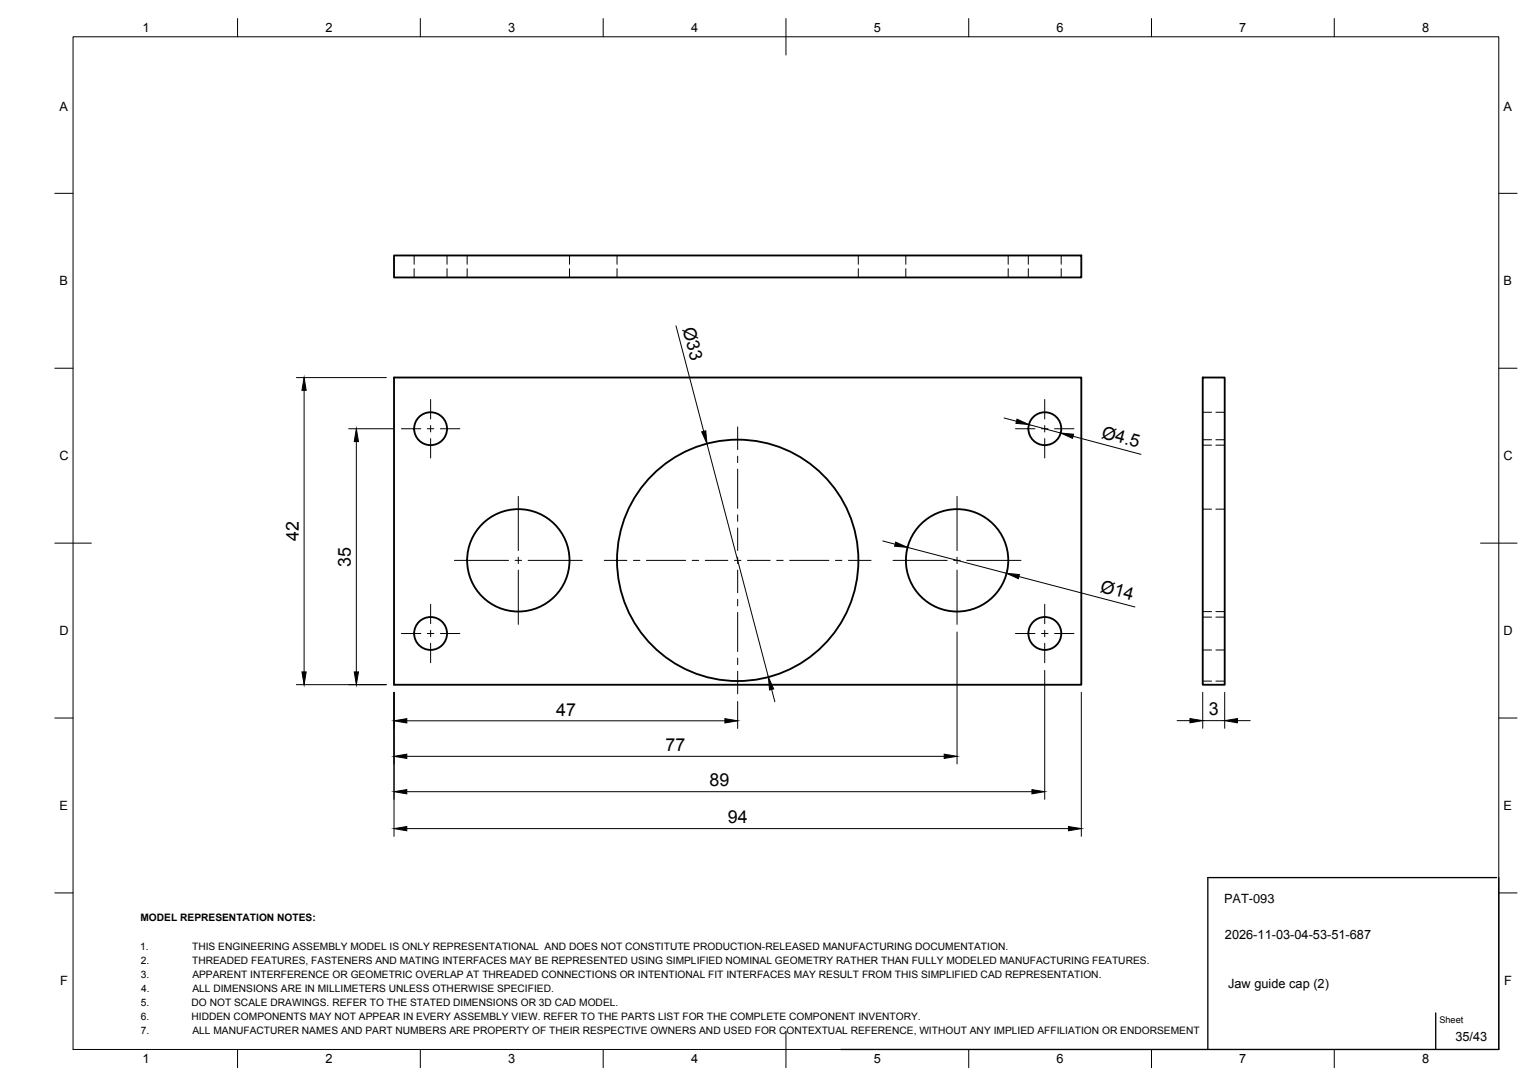
ISO-10303-21;
HEADER;
/* Generated by software containing ST-Developer
 * from STEP Tools, Inc. (www.steptools.com) 
 */

FILE_DESCRIPTION(
/* description */ ('Self-centering screw clamp'),
/* implementation_level */ '2;1');

FILE_NAME(
/* name */ 'Jaw guide cap (2).step',
/* time_stamp */ '2026-10-28T03:25:31-07:00',
/* author */ (''),
/* organization */ (''),
/* preprocessor_version */ 'ST-DEVELOPER v20.2',
/* originating_system */ 'Autodesk Translation Framework v15.17.0.0',
/* authorisation */ '');

FILE_SCHEMA (('AUTOMOTIVE_DESIGN { 1 0 10303 214 3 1 1 }'));
ENDSEC;

DATA;
#10=MECHANICAL_DESIGN_GEOMETRIC_PRESENTATION_REPRESENTATION('',(#656),#16799);
#567=SHAPE_REPRESENTATION_RELATIONSHIP('SRR','None',#17043,#608);
#608=ADVANCED_BREP_SHAPE_REPRESENTATION('',(#704),#16781);
#656=STYLED_ITEM('',(#17312),#704);
#704=MANIFOLD_SOLID_BREP('Body1',#9107);
#936=FACE_BOUND('',#2337,.T.);
#937=FACE_BOUND('',#2338,.T.);
#938=FACE_BOUND('',#2339,.T.);
#939=FACE_BOUND('',#2340,.T.);
#940=FACE_BOUND('',#2341,.T.);
#941=FACE_BOUND('',#2342,.T.);
#942=FACE_BOUND('',#2343,.T.);
#943=FACE_BOUND('',#2346,.T.);
#944=FACE_BOUND('',#2347,.T.);
#945=FACE_BOUND('',#2348,.T.);
#946=FACE_BOUND('',#2349,.T.);
#947=FACE_BOUND('',#2350,.T.);
#948=FACE_BOUND('',#2351,.T.);
#949=FACE_BOUND('',#2352,.T.);
#1173=PLANE('',#10330);
#1174=PLANE('',#10331);
#1175=PLANE('',#10332);
#1176=PLANE('',#10333);
#1177=PLANE('',#10334);
#1178=PLANE('',#10335);
#1606=FACE_OUTER_BOUND('',#2328,.T.);
#1607=FACE_OUTER_BOUND('',#2329,.T.);
#1608=FACE_OUTER_BOUND('',#2330,.T.);
#1609=FACE_OUTER_BOUND('',#2331,.T.);
#1610=FACE_OUTER_BOUND('',#2332,.T.);
#1611=FACE_OUTER_BOUND('',#2333,.T.);
#1612=FACE_OUTER_BOUND('',#2334,.T.);
#1613=FACE_OUTER_BOUND('',#2335,.T.);
#1614=FACE_OUTER_BOUND('',#2336,.T.);
#1615=FACE_OUTER_BOUND('',#2344,.T.);
#1616=FACE_OUTER_BOUND('',#2345,.T.);
#1617=FACE_OUTER_BOUND('',#2353,.T.);
#1618=FACE_OUTER_BOUND('',#2354,.T.);
#2328=EDGE_LOOP('',(#7653,#7654,#7655,#7656));
#2329=EDGE_LOOP('',(#7657,#7658,#7659,#7660));
#2330=EDGE_LOOP('',(#7661,#7662,#7663,#7664));
#2331=EDGE_LOOP('',(#7665,#7666,#7667,#7668));
#2332=EDGE_LOOP('',(#7669,#7670,#7671,#7672));
#2333=EDGE_LOOP('',(#7673,#7674,#7675,#7676));
#2334=EDGE_LOOP('',(#7677,#7678,#7679,#7680));
#2335=EDGE_LOOP('',(#7681,#7682,#7683,#7684));
#2336=EDGE_LOOP('',(#7685,#7686,#7687,#7688));
#2337=EDGE_LOOP('',(#7689));
#2338=EDGE_LOOP('',(#7690));
#2339=EDGE_LOOP('',(#7691));
#2340=EDGE_LOOP('',(#7692));
#2341=EDGE_LOOP('',(#7693));
#2342=EDGE_LOOP('',(#7694));
#2343=EDGE_LOOP('',(#7695));
#2344=EDGE_LOOP('',(#7696,#7697,#7698,#7699));
#2345=EDGE_LOOP('',(#7700,#7701,#7702,#7703));
#2346=EDGE_LOOP('',(#7704));
#2347=EDGE_LOOP('',(#7705));
#2348=EDGE_LOOP('',(#7706));
#2349=EDGE_LOOP('',(#7707));
#2350=EDGE_LOOP('',(#7708));
#2351=EDGE_LOOP('',(#7709));
#2352=EDGE_LOOP('',(#7710));
#2353=EDGE_LOOP('',(#7711,#7712,#7713,#7714));
#2354=EDGE_LOOP('',(#7715,#7716,#7717,#7718));
#2959=LINE('',#15709,#3532);
#2960=LINE('',#15715,#3533);
#2961=LINE('',#15721,#3534);
#2962=LINE('',#15727,#3535);
#2963=LINE('',#15733,#3536);
#2964=LINE('',#15739,#3537);
#2965=LINE('',#15745,#3538);
#2966=LINE('',#15750,#3539);
#2967=LINE('',#15752,#3540);
#2968=LINE('',#15754,#3541);
#2969=LINE('',#15755,#3542);
#2970=LINE('',#15758,#3543);
#2971=LINE('',#15760,#3544);
#2972=LINE('',#15761,#3545);
#2973=LINE('',#15764,#3546);
#2974=LINE('',#15766,#3547);
#2975=LINE('',#15767,#3548);
#2976=LINE('',#15769,#3549);
#2977=LINE('',#15770,#3550);
#3532=VECTOR('',#12602,0.225);
#3533=VECTOR('',#12609,0.225);
#3534=VECTOR('',#12616,0.225);
#3535=VECTOR('',#12623,0.225);
#3536=VECTOR('',#12630,1.65);
#3537=VECTOR('',#12637,0.7);
#3538=VECTOR('',#12644,0.7);
#3539=VECTOR('',#12649,1.);
#3540=VECTOR('',#12650,1.);
#3541=VECTOR('',#12651,1.);
#3542=VECTOR('',#12652,1.);
#3543=VECTOR('',#12655,1.);
#3544=VECTOR('',#12656,1.);
#3545=VECTOR('',#12657,1.);
#3546=VECTOR('',#12660,1.);
#3547=VECTOR('',#12661,1.);
#3548=VECTOR('',#12662,1.);
#3549=VECTOR('',#12665,1.);
#3550=VECTOR('',#12666,1.);
#4086=CIRCLE('',#10310,0.225);
#4087=CIRCLE('',#10311,0.225);
#4088=CIRCLE('',#10313,0.225);
#4089=CIRCLE('',#10314,0.225);
#4090=CIRCLE('',#10316,0.225);
#4091=CIRCLE('',#10317,0.225);
#4092=CIRCLE('',#10319,0.225);
#4093=CIRCLE('',#10320,0.225);
#4094=CIRCLE('',#10322,1.65);
#4095=CIRCLE('',#10323,1.65);
#4096=CIRCLE('',#10325,0.7);
#4097=CIRCLE('',#10326,0.7);
#4098=CIRCLE('',#10328,0.7);
#4099=CIRCLE('',#10329,0.7);
#4745=VERTEX_POINT('',#15706);
#4746=VERTEX_POINT('',#15708);
#4747=VERTEX_POINT('',#15712);
#4748=VERTEX_POINT('',#15714);
#4749=VERTEX_POINT('',#15718);
#4750=VERTEX_POINT('',#15720);
#4751=VERTEX_POINT('',#15724);
#4752=VERTEX_POINT('',#15726);
#4753=VERTEX_POINT('',#15730);
#4754=VERTEX_POINT('',#15732);
#4755=VERTEX_POINT('',#15736);
#4756=VERTEX_POINT('',#15738);
#4757=VERTEX_POINT('',#15742);
#4758=VERTEX_POINT('',#15744);
#4759=VERTEX_POINT('',#15748);
#4760=VERTEX_POINT('',#15749);
#4761=VERTEX_POINT('',#15751);
#4762=VERTEX_POINT('',#15753);
#4763=VERTEX_POINT('',#15757);
#4764=VERTEX_POINT('',#15759);
#4765=VERTEX_POINT('',#15763);
#4766=VERTEX_POINT('',#15765);
#5751=EDGE_CURVE('',#4745,#4745,#4086,.T.);
#5752=EDGE_CURVE('',#4745,#4746,#2959,.T.);
#5753=EDGE_CURVE('',#4746,#4746,#4087,.T.);
#5754=EDGE_CURVE('',#4747,#4747,#4088,.T.);
#5755=EDGE_CURVE('',#4747,#4748,#2960,.T.);
#5756=EDGE_CURVE('',#4748,#4748,#4089,.T.);
#5757=EDGE_CURVE('',#4749,#4749,#4090,.T.);
#5758=EDGE_CURVE('',#4749,#4750,#2961,.T.);
#5759=EDGE_CURVE('',#4750,#4750,#4091,.T.);
#5760=EDGE_CURVE('',#4751,#4751,#4092,.T.);
#5761=EDGE_CURVE('',#4751,#4752,#2962,.T.);
#5762=EDGE_CURVE('',#4752,#4752,#4093,.T.);
#5763=EDGE_CURVE('',#4753,#4753,#4094,.T.);
#5764=EDGE_CURVE('',#4753,#4754,#2963,.T.);
#5765=EDGE_CURVE('',#4754,#4754,#4095,.T.);
#5766=EDGE_CURVE('',#4755,#4755,#4096,.T.);
#5767=EDGE_CURVE('',#4755,#4756,#2964,.T.);
#5768=EDGE_CURVE('',#4756,#4756,#4097,.T.);
#5769=EDGE_CURVE('',#4757,#4757,#4098,.T.);
#5770=EDGE_CURVE('',#4757,#4758,#2965,.T.);
#5771=EDGE_CURVE('',#4758,#4758,#4099,.T.);
#5772=EDGE_CURVE('',#4759,#4760,#2966,.T.);
#5773=EDGE_CURVE('',#4760,#4761,#2967,.T.);
#5774=EDGE_CURVE('',#4762,#4761,#2968,.T.);
#5775=EDGE_CURVE('',#4759,#4762,#2969,.T.);
#5776=EDGE_CURVE('',#4763,#4759,#2970,.T.);
#5777=EDGE_CURVE('',#4764,#4762,#2971,.T.);
#5778=EDGE_CURVE('',#4763,#4764,#2972,.T.);
#5779=EDGE_CURVE('',#4765,#4763,#2973,.T.);
#5780=EDGE_CURVE('',#4766,#4764,#2974,.T.);
#5781=EDGE_CURVE('',#4765,#4766,#2975,.T.);
#5782=EDGE_CURVE('',#4760,#4765,#2976,.T.);
#5783=EDGE_CURVE('',#4761,#4766,#2977,.T.);
#7653=ORIENTED_EDGE('',*,*,#5751,.F.);
#7654=ORIENTED_EDGE('',*,*,#5752,.T.);
#7655=ORIENTED_EDGE('',*,*,#5753,.F.);
#7656=ORIENTED_EDGE('',*,*,#5752,.F.);
#7657=ORIENTED_EDGE('',*,*,#5754,.F.);
#7658=ORIENTED_EDGE('',*,*,#5755,.T.);
#7659=ORIENTED_EDGE('',*,*,#5756,.F.);
#7660=ORIENTED_EDGE('',*,*,#5755,.F.);
#7661=ORIENTED_EDGE('',*,*,#5757,.F.);
#7662=ORIENTED_EDGE('',*,*,#5758,.T.);
#7663=ORIENTED_EDGE('',*,*,#5759,.F.);
#7664=ORIENTED_EDGE('',*,*,#5758,.F.);
#7665=ORIENTED_EDGE('',*,*,#5760,.F.);
#7666=ORIENTED_EDGE('',*,*,#5761,.T.);
#7667=ORIENTED_EDGE('',*,*,#5762,.F.);
#7668=ORIENTED_EDGE('',*,*,#5761,.F.);
#7669=ORIENTED_EDGE('',*,*,#5763,.F.);
#7670=ORIENTED_EDGE('',*,*,#5764,.T.);
#7671=ORIENTED_EDGE('',*,*,#5765,.F.);
#7672=ORIENTED_EDGE('',*,*,#5764,.F.);
#7673=ORIENTED_EDGE('',*,*,#5766,.F.);
#7674=ORIENTED_EDGE('',*,*,#5767,.T.);
#7675=ORIENTED_EDGE('',*,*,#5768,.F.);
#7676=ORIENTED_EDGE('',*,*,#5767,.F.);
#7677=ORIENTED_EDGE('',*,*,#5769,.F.);
#7678=ORIENTED_EDGE('',*,*,#5770,.T.);
#7679=ORIENTED_EDGE('',*,*,#5771,.F.);
#7680=ORIENTED_EDGE('',*,*,#5770,.F.);
#7681=ORIENTED_EDGE('',*,*,#5772,.T.);
#7682=ORIENTED_EDGE('',*,*,#5773,.T.);
#7683=ORIENTED_EDGE('',*,*,#5774,.F.);
#7684=ORIENTED_EDGE('',*,*,#5775,.F.);
#7685=ORIENTED_EDGE('',*,*,#5776,.T.);
#7686=ORIENTED_EDGE('',*,*,#5775,.T.);
#7687=ORIENTED_EDGE('',*,*,#5777,.F.);
#7688=ORIENTED_EDGE('',*,*,#5778,.F.);
#7689=ORIENTED_EDGE('',*,*,#5771,.T.);
#7690=ORIENTED_EDGE('',*,*,#5768,.T.);
#7691=ORIENTED_EDGE('',*,*,#5765,.T.);
#7692=ORIENTED_EDGE('',*,*,#5762,.T.);
#7693=ORIENTED_EDGE('',*,*,#5759,.T.);
#7694=ORIENTED_EDGE('',*,*,#5756,.T.);
#7695=ORIENTED_EDGE('',*,*,#5753,.T.);
#7696=ORIENTED_EDGE('',*,*,#5779,.T.);
#7697=ORIENTED_EDGE('',*,*,#5778,.T.);
#7698=ORIENTED_EDGE('',*,*,#5780,.F.);
#7699=ORIENTED_EDGE('',*,*,#5781,.F.);
#7700=ORIENTED_EDGE('',*,*,#5782,.T.);
#7701=ORIENTED_EDGE('',*,*,#5781,.T.);
#7702=ORIENTED_EDGE('',*,*,#5783,.F.);
#7703=ORIENTED_EDGE('',*,*,#5773,.F.);
#7704=ORIENTED_EDGE('',*,*,#5769,.T.);
#7705=ORIENTED_EDGE('',*,*,#5766,.T.);
#7706=ORIENTED_EDGE('',*,*,#5763,.T.);
#7707=ORIENTED_EDGE('',*,*,#5760,.T.);
#7708=ORIENTED_EDGE('',*,*,#5757,.T.);
#7709=ORIENTED_EDGE('',*,*,#5754,.T.);
#7710=ORIENTED_EDGE('',*,*,#5751,.T.);
#7711=ORIENTED_EDGE('',*,*,#5783,.T.);
#7712=ORIENTED_EDGE('',*,*,#5780,.T.);
#7713=ORIENTED_EDGE('',*,*,#5777,.T.);
#7714=ORIENTED_EDGE('',*,*,#5774,.T.);
#7715=ORIENTED_EDGE('',*,*,#5782,.F.);
#7716=ORIENTED_EDGE('',*,*,#5772,.F.);
#7717=ORIENTED_EDGE('',*,*,#5776,.F.);
#7718=ORIENTED_EDGE('',*,*,#5779,.F.);
#8509=CYLINDRICAL_SURFACE('',#10309,0.225);
#8510=CYLINDRICAL_SURFACE('',#10312,0.225);
#8511=CYLINDRICAL_SURFACE('',#10315,0.225);
#8512=CYLINDRICAL_SURFACE('',#10318,0.225);
#8513=CYLINDRICAL_SURFACE('',#10321,1.65);
#8514=CYLINDRICAL_SURFACE('',#10324,0.7);
#8515=CYLINDRICAL_SURFACE('',#10327,0.7);
#8904=ADVANCED_FACE('',(#1606),#8509,.F.);
#8905=ADVANCED_FACE('',(#1607),#8510,.F.);
#8906=ADVANCED_FACE('',(#1608),#8511,.F.);
#8907=ADVANCED_FACE('',(#1609),#8512,.F.);
#8908=ADVANCED_FACE('',(#1610),#8513,.F.);
#8909=ADVANCED_FACE('',(#1611),#8514,.F.);
#8910=ADVANCED_FACE('',(#1612),#8515,.F.);
#8911=ADVANCED_FACE('',(#1613),#1173,.T.);
#8912=ADVANCED_FACE('',(#1614,#936,#937,#938,#939,#940,#941,#942),#1174,
 .T.);
#8913=ADVANCED_FACE('',(#1615),#1175,.T.);
#8914=ADVANCED_FACE('',(#1616,#943,#944,#945,#946,#947,#948,#949),#1176,
 .T.);
#8915=ADVANCED_FACE('',(#1617),#1177,.T.);
#8916=ADVANCED_FACE('',(#1618),#1178,.F.);
#9107=CLOSED_SHELL('',(#8904,#8905,#8906,#8907,#8908,#8909,#8910,#8911,
#8912,#8913,#8914,#8915,#8916));
#10308=AXIS2_PLACEMENT_3D('',#15704,#12596,#12597);
#10309=AXIS2_PLACEMENT_3D('',#15705,#12598,#12599);
#10310=AXIS2_PLACEMENT_3D('',#15707,#12600,#12601);
#10311=AXIS2_PLACEMENT_3D('',#15710,#12603,#12604);
#10312=AXIS2_PLACEMENT_3D('',#15711,#12605,#12606);
#10313=AXIS2_PLACEMENT_3D('',#15713,#12607,#12608);
#10314=AXIS2_PLACEMENT_3D('',#15716,#12610,#12611);
#10315=AXIS2_PLACEMENT_3D('',#15717,#12612,#12613);
#10316=AXIS2_PLACEMENT_3D('',#15719,#12614,#12615);
#10317=AXIS2_PLACEMENT_3D('',#15722,#12617,#12618);
#10318=AXIS2_PLACEMENT_3D('',#15723,#12619,#12620);
#10319=AXIS2_PLACEMENT_3D('',#15725,#12621,#12622);
#10320=AXIS2_PLACEMENT_3D('',#15728,#12624,#12625);
#10321=AXIS2_PLACEMENT_3D('',#15729,#12626,#12627);
#10322=AXIS2_PLACEMENT_3D('',#15731,#12628,#12629);
#10323=AXIS2_PLACEMENT_3D('',#15734,#12631,#12632);
#10324=AXIS2_PLACEMENT_3D('',#15735,#12633,#12634);
#10325=AXIS2_PLACEMENT_3D('',#15737,#12635,#12636);
#10326=AXIS2_PLACEMENT_3D('',#15740,#12638,#12639);
#10327=AXIS2_PLACEMENT_3D('',#15741,#12640,#12641);
#10328=AXIS2_PLACEMENT_3D('',#15743,#12642,#12643);
#10329=AXIS2_PLACEMENT_3D('',#15746,#12645,#12646);
#10330=AXIS2_PLACEMENT_3D('',#15747,#12647,#12648);
#10331=AXIS2_PLACEMENT_3D('',#15756,#12653,#12654);
#10332=AXIS2_PLACEMENT_3D('',#15762,#12658,#12659);
#10333=AXIS2_PLACEMENT_3D('',#15768,#12663,#12664);
#10334=AXIS2_PLACEMENT_3D('',#15771,#12667,#12668);
#10335=AXIS2_PLACEMENT_3D('',#15772,#12669,#12670);
#12596=DIRECTION('axis',(0.,0.,1.));
#12597=DIRECTION('refdir',(1.,0.,0.));
#12598=DIRECTION('center_axis',(1.,0.,0.));
#12599=DIRECTION('ref_axis',(0.,0.,-1.));
#12600=DIRECTION('center_axis',(1.,0.,0.));
#12601=DIRECTION('ref_axis',(0.,0.,-1.));
#12602=DIRECTION('',(1.,0.,0.));
#12603=DIRECTION('center_axis',(-1.,0.,0.));
#12604=DIRECTION('ref_axis',(0.,0.,-1.));
#12605=DIRECTION('center_axis',(1.,0.,0.));
#12606=DIRECTION('ref_axis',(0.,0.,-1.));
#12607=DIRECTION('center_axis',(1.,0.,0.));
#12608=DIRECTION('ref_axis',(0.,0.,-1.));
#12609=DIRECTION('',(1.,0.,0.));
#12610=DIRECTION('center_axis',(-1.,0.,0.));
#12611=DIRECTION('ref_axis',(0.,0.,-1.));
#12612=DIRECTION('center_axis',(1.,0.,0.));
#12613=DIRECTION('ref_axis',(0.,0.,-1.));
#12614=DIRECTION('center_axis',(1.,0.,0.));
#12615=DIRECTION('ref_axis',(0.,0.,-1.));
#12616=DIRECTION('',(1.,0.,0.));
#12617=DIRECTION('center_axis',(-1.,0.,0.));
#12618=DIRECTION('ref_axis',(0.,0.,-1.));
#12619=DIRECTION('center_axis',(1.,0.,0.));
#12620=DIRECTION('ref_axis',(0.,0.,-1.));
#12621=DIRECTION('center_axis',(1.,0.,0.));
#12622=DIRECTION('ref_axis',(0.,0.,-1.));
#12623=DIRECTION('',(1.,0.,0.));
#12624=DIRECTION('center_axis',(-1.,0.,0.));
#12625=DIRECTION('ref_axis',(0.,0.,-1.));
#12626=DIRECTION('center_axis',(1.,0.,0.));
#12627=DIRECTION('ref_axis',(0.,0.,-1.));
#12628=DIRECTION('center_axis',(1.,0.,0.));
#12629=DIRECTION('ref_axis',(0.,0.,-1.));
#12630=DIRECTION('',(1.,0.,0.));
#12631=DIRECTION('center_axis',(-1.,0.,0.));
#12632=DIRECTION('ref_axis',(0.,0.,-1.));
#12633=DIRECTION('center_axis',(1.,0.,0.));
#12634=DIRECTION('ref_axis',(0.,0.,-1.));
#12635=DIRECTION('center_axis',(1.,0.,0.));
#12636=DIRECTION('ref_axis',(0.,0.,-1.));
#12637=DIRECTION('',(1.,0.,0.));
#12638=DIRECTION('center_axis',(-1.,0.,0.));
#12639=DIRECTION('ref_axis',(0.,0.,-1.));
#12640=DIRECTION('center_axis',(1.,0.,0.));
#12641=DIRECTION('ref_axis',(0.,0.,-1.));
#12642=DIRECTION('center_axis',(1.,0.,0.));
#12643=DIRECTION('ref_axis',(0.,0.,-1.));
#12644=DIRECTION('',(1.,0.,0.));
#12645=DIRECTION('center_axis',(-1.,0.,0.));
#12646=DIRECTION('ref_axis',(0.,0.,-1.));
#12647=DIRECTION('center_axis',(0.,1.,0.));
#12648=DIRECTION('ref_axis',(-1.,0.,0.));
#12649=DIRECTION('',(-1.,0.,0.));
#12650=DIRECTION('',(0.,0.,1.));
#12651=DIRECTION('',(-1.,0.,0.));
#12652=DIRECTION('',(0.,0.,1.));
#12653=DIRECTION('center_axis',(1.,0.,0.));
#12654=DIRECTION('ref_axis',(0.,1.,0.));
#12655=DIRECTION('',(0.,1.,0.));
#12656=DIRECTION('',(0.,1.,0.));
#12657=DIRECTION('',(0.,0.,1.));
#12658=DIRECTION('center_axis',(0.,-1.,0.));
#12659=DIRECTION('ref_axis',(1.,0.,0.));
#12660=DIRECTION('',(1.,0.,0.));
#12661=DIRECTION('',(1.,0.,0.));
#12662=DIRECTION('',(0.,0.,1.));
#12663=DIRECTION('center_axis',(-1.,0.,0.));
#12664=DIRECTION('ref_axis',(0.,-1.,0.));
#12665=DIRECTION('',(0.,-1.,0.));
#12666=DIRECTION('',(0.,-1.,0.));
#12667=DIRECTION('center_axis',(0.,0.,1.));
#12668=DIRECTION('ref_axis',(1.,0.,0.));
#12669=DIRECTION('center_axis',(0.,0.,1.));
#12670=DIRECTION('ref_axis',(1.,0.,0.));
#15704=CARTESIAN_POINT('',(0.,0.,0.));
#15705=CARTESIAN_POINT('Origin',(5.1,4.2,3.));
#15706=CARTESIAN_POINT('',(5.2,4.2,3.225));
#15707=CARTESIAN_POINT('Origin',(5.2,4.2,3.));
#15708=CARTESIAN_POINT('',(5.5,4.2,3.225));
#15709=CARTESIAN_POINT('',(5.1,4.2,3.225));
#15710=CARTESIAN_POINT('Origin',(5.5,4.2,3.));
#15711=CARTESIAN_POINT('Origin',(5.1,-4.2,5.8));
#15712=CARTESIAN_POINT('',(5.2,-4.2,6.025));
#15713=CARTESIAN_POINT('Origin',(5.2,-4.2,5.8));
#15714=CARTESIAN_POINT('',(5.5,-4.2,6.025));
#15715=CARTESIAN_POINT('',(5.1,-4.2,6.025));
#15716=CARTESIAN_POINT('Origin',(5.5,-4.2,5.8));
#15717=CARTESIAN_POINT('Origin',(5.1,-4.2,3.));
#15718=CARTESIAN_POINT('',(5.2,-4.2,3.225));
#15719=CARTESIAN_POINT('Origin',(5.2,-4.2,3.));
#15720=CARTESIAN_POINT('',(5.5,-4.2,3.225));
#15721=CARTESIAN_POINT('',(5.1,-4.2,3.225));
#15722=CARTESIAN_POINT('Origin',(5.5,-4.2,3.));
#15723=CARTESIAN_POINT('Origin',(5.1,4.2,5.8));
#15724=CARTESIAN_POINT('',(5.2,4.2,6.025));
#15725=CARTESIAN_POINT('Origin',(5.2,4.2,5.8));
#15726=CARTESIAN_POINT('',(5.5,4.2,6.025));
#15727=CARTESIAN_POINT('',(5.1,4.2,6.025));
#15728=CARTESIAN_POINT('Origin',(5.5,4.2,5.8));
#15729=CARTESIAN_POINT('Origin',(5.1,0.,4.));
#15730=CARTESIAN_POINT('',(5.2,-2.02066721859313E-16,5.65));
#15731=CARTESIAN_POINT('Origin',(5.2,0.,4.));
#15732=CARTESIAN_POINT('',(5.5,2.02066721859313E-16,5.65));
#15733=CARTESIAN_POINT('',(5.1,-2.02066721859313E-16,5.65));
#15734=CARTESIAN_POINT('Origin',(5.5,0.,4.));
#15735=CARTESIAN_POINT('Origin',(5.1,-3.,4.));
#15736=CARTESIAN_POINT('',(5.2,-3.,4.7));
#15737=CARTESIAN_POINT('Origin',(5.2,-3.,4.));
#15738=CARTESIAN_POINT('',(5.5,-3.,4.7));
#15739=CARTESIAN_POINT('',(5.1,-3.,4.7));
#15740=CARTESIAN_POINT('Origin',(5.5,-3.,4.));
#15741=CARTESIAN_POINT('Origin',(5.1,3.,4.));
#15742=CARTESIAN_POINT('',(5.2,3.,4.7));
#15743=CARTESIAN_POINT('Origin',(5.2,3.,4.));
#15744=CARTESIAN_POINT('',(5.5,3.,4.7));
#15745=CARTESIAN_POINT('',(5.1,3.,4.7));
#15746=CARTESIAN_POINT('Origin',(5.5,3.,4.));
#15747=CARTESIAN_POINT('Origin',(5.5,4.7,2.3));
#15748=CARTESIAN_POINT('',(5.5,4.7,2.3));
#15749=CARTESIAN_POINT('',(5.2,4.7,2.3));
#15750=CARTESIAN_POINT('',(5.5,4.7,2.3));
#15751=CARTESIAN_POINT('',(5.2,4.7,6.5));
#15752=CARTESIAN_POINT('',(5.2,4.7,2.3));
#15753=CARTESIAN_POINT('',(5.5,4.7,6.5));
#15754=CARTESIAN_POINT('',(5.5,4.7,6.5));
#15755=CARTESIAN_POINT('',(5.5,4.7,2.3));
#15756=CARTESIAN_POINT('Origin',(5.5,-4.7,2.3));
#15757=CARTESIAN_POINT('',(5.5,-4.7,2.3));
#15758=CARTESIAN_POINT('',(5.5,-4.7,2.3));
#15759=CARTESIAN_POINT('',(5.5,-4.7,6.5));
#15760=CARTESIAN_POINT('',(5.5,-4.7,6.5));
#15761=CARTESIAN_POINT('',(5.5,-4.7,2.3));
#15762=CARTESIAN_POINT('Origin',(5.2,-4.7,2.3));
#15763=CARTESIAN_POINT('',(5.2,-4.7,2.3));
#15764=CARTESIAN_POINT('',(5.2,-4.7,2.3));
#15765=CARTESIAN_POINT('',(5.2,-4.7,6.5));
#15766=CARTESIAN_POINT('',(5.2,-4.7,6.5));
#15767=CARTESIAN_POINT('',(5.2,-4.7,2.3));
#15768=CARTESIAN_POINT('Origin',(5.2,4.7,2.3));
#15769=CARTESIAN_POINT('',(5.2,4.7,2.3));
#15770=CARTESIAN_POINT('',(5.2,4.7,6.5));
#15771=CARTESIAN_POINT('Origin',(5.35,0.,6.5));
#15772=CARTESIAN_POINT('Origin',(5.35,0.,2.3));
#16732=UNCERTAINTY_MEASURE_WITH_UNIT(LENGTH_MEASURE(0.001),#16800,
'DISTANCE_ACCURACY_VALUE',
'Maximum model space distance between geometric entities at asserted c
onnectivities');
#16750=UNCERTAINTY_MEASURE_WITH_UNIT(LENGTH_MEASURE(0.001),#16800,
'DISTANCE_ACCURACY_VALUE',
'Maximum model space distance between geometric entities at asserted c
onnectivities');
#16781=(
GEOMETRIC_REPRESENTATION_CONTEXT(3)
GLOBAL_UNCERTAINTY_ASSIGNED_CONTEXT((#16732))
GLOBAL_UNIT_ASSIGNED_CONTEXT((#16800,#16802,#16803))
REPRESENTATION_CONTEXT('','3D')
);
#16799=(
GEOMETRIC_REPRESENTATION_CONTEXT(3)
GLOBAL_UNCERTAINTY_ASSIGNED_CONTEXT((#16750))
GLOBAL_UNIT_ASSIGNED_CONTEXT((#16800,#16802,#16803))
REPRESENTATION_CONTEXT('','3D')
);
#16800=(
LENGTH_UNIT()
NAMED_UNIT(*)
SI_UNIT(.CENTI.,.METRE.)
);
#16802=(
NAMED_UNIT(*)
PLANE_ANGLE_UNIT()
SI_UNIT($,.RADIAN.)
);
#16803=(
NAMED_UNIT(*)
SI_UNIT($,.STERADIAN.)
SOLID_ANGLE_UNIT()
);
#16834=SHAPE_DEFINITION_REPRESENTATION(#16887,#17043);
#16887=PRODUCT_DEFINITION_SHAPE('',$,#17092);
#17043=SHAPE_REPRESENTATION('',(#10308),#16781);
#17061=PRODUCT_DEFINITION_CONTEXT('part definition',#17207,'design');
#17092=PRODUCT_DEFINITION('Jaw guide cap (2)','Jaw guide cap (2)',#17140,
#17061);
#17140=PRODUCT_DEFINITION_FORMATION('',$,#17239);
#17207=APPLICATION_CONTEXT(
'Core Data for Automotive Mechanical Design Process');
#17208=PRODUCT_CONTEXT('part definition',#17207,'mechanical');
#17239=PRODUCT('Jaw guide cap (2)','Jaw guide cap (2)','Jaw guide cap (2)',(#17208));
#17306=COLOUR_RGB('Light Blue',0.38,0.62,0.78);
#17307=FILL_AREA_STYLE_COLOUR('',#17306);
#17308=FILL_AREA_STYLE('',(#17307));
#17309=SURFACE_STYLE_FILL_AREA(#17308);
#17310=SURFACE_SIDE_STYLE('',(#17309));
#17311=SURFACE_STYLE_USAGE(.BOTH.,#17310);
#17312=PRESENTATION_STYLE_ASSIGNMENT((#17311));
ENDSEC;
END-ISO-10303-21;
